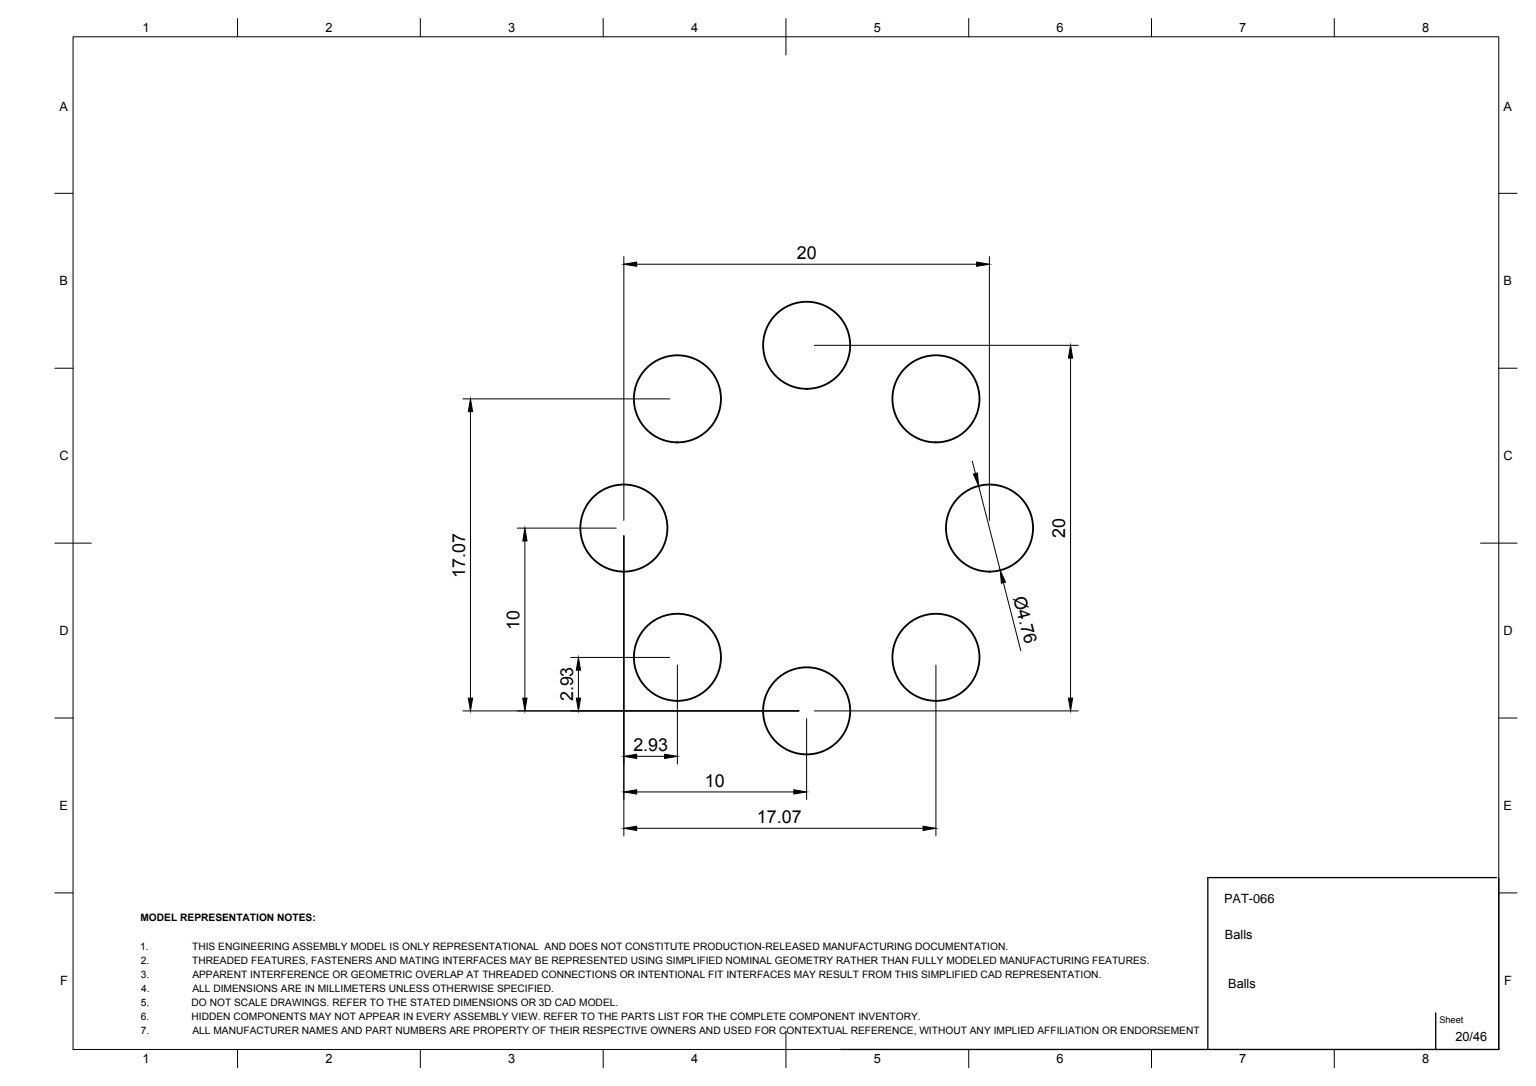
ISO-10303-21;
HEADER;
/* Generated by software containing ST-Developer
 * from STEP Tools, Inc. (www.steptools.com) 
 */

FILE_DESCRIPTION(
/* description */ ('Lever-operated bar clamp (toggle)'),
/* implementation_level */ '2;1');

FILE_NAME(
/* name */ 'Balls.step',
/* time_stamp */ '2026-10-28T03:25:02-07:00',
/* author */ (''),
/* organization */ (''),
/* preprocessor_version */ 'ST-DEVELOPER v20.2',
/* originating_system */ 'Autodesk Translation Framework v15.17.0.0',
/* authorisation */ '');

FILE_SCHEMA (('AUTOMOTIVE_DESIGN { 1 0 10303 214 3 1 1 }'));
ENDSEC;

DATA;
#10=MECHANICAL_DESIGN_GEOMETRIC_PRESENTATION_REPRESENTATION('',(#424,#425,#426,#427,#428,#429,#430,#431),#12413);
#287=SPHERICAL_SURFACE('',#7369,0.23815);
#288=SPHERICAL_SURFACE('',#7371,0.23815);
#289=SPHERICAL_SURFACE('',#7373,0.23815);
#290=SPHERICAL_SURFACE('',#7375,0.23815);
#291=SPHERICAL_SURFACE('',#7377,0.23815);
#292=SPHERICAL_SURFACE('',#7379,0.23815);
#293=SPHERICAL_SURFACE('',#7381,0.23815);
#294=SPHERICAL_SURFACE('',#7383,0.23815);
#348=SHAPE_REPRESENTATION_RELATIONSHIP('SRR','None',#12588,#386);
#386=ADVANCED_BREP_SHAPE_REPRESENTATION('',(#470,#471,#472,#473,#474,#475,
#476,#477),#12385);
#424=STYLED_ITEM('',(#12869),#470);
#425=STYLED_ITEM('',(#12869),#471);
#426=STYLED_ITEM('',(#12869),#472);
#427=STYLED_ITEM('',(#12869),#473);
#428=STYLED_ITEM('',(#12869),#474);
#429=STYLED_ITEM('',(#12869),#475);
#430=STYLED_ITEM('',(#12869),#476);
#431=STYLED_ITEM('',(#12869),#477);
#470=MANIFOLD_SOLID_BREP('Body1',#6584);
#471=MANIFOLD_SOLID_BREP('Body2',#6585);
#472=MANIFOLD_SOLID_BREP('Body3',#6586);
#473=MANIFOLD_SOLID_BREP('Body4',#6587);
#474=MANIFOLD_SOLID_BREP('Body5',#6588);
#475=MANIFOLD_SOLID_BREP('Body6',#6589);
#476=MANIFOLD_SOLID_BREP('Body7',#6590);
#477=MANIFOLD_SOLID_BREP('Body8',#6591);
#1055=FACE_OUTER_BOUND('',#1553,.T.);
#1056=FACE_OUTER_BOUND('',#1554,.T.);
#1057=FACE_OUTER_BOUND('',#1555,.T.);
#1058=FACE_OUTER_BOUND('',#1556,.T.);
#1059=FACE_OUTER_BOUND('',#1557,.T.);
#1060=FACE_OUTER_BOUND('',#1558,.T.);
#1061=FACE_OUTER_BOUND('',#1559,.T.);
#1062=FACE_OUTER_BOUND('',#1560,.T.);
#1553=EDGE_LOOP('',(#5109,#5110));
#1554=EDGE_LOOP('',(#5111,#5112));
#1555=EDGE_LOOP('',(#5113,#5114));
#1556=EDGE_LOOP('',(#5115,#5116));
#1557=EDGE_LOOP('',(#5117,#5118));
#1558=EDGE_LOOP('',(#5119,#5120));
#1559=EDGE_LOOP('',(#5121,#5122));
#1560=EDGE_LOOP('',(#5123,#5124));
#2878=CIRCLE('',#7370,0.23815);
#2879=CIRCLE('',#7372,0.23815);
#2880=CIRCLE('',#7374,0.23815);
#2881=CIRCLE('',#7376,0.23815);
#2882=CIRCLE('',#7378,0.23815);
#2883=CIRCLE('',#7380,0.23815);
#2884=CIRCLE('',#7382,0.23815);
#2885=CIRCLE('',#7384,0.23815);
#3301=VERTEX_POINT('',#10802);
#3302=VERTEX_POINT('',#10803);
#3303=VERTEX_POINT('',#10806);
#3304=VERTEX_POINT('',#10807);
#3305=VERTEX_POINT('',#10810);
#3306=VERTEX_POINT('',#10811);
#3307=VERTEX_POINT('',#10814);
#3308=VERTEX_POINT('',#10815);
#3309=VERTEX_POINT('',#10818);
#3310=VERTEX_POINT('',#10819);
#3311=VERTEX_POINT('',#10822);
#3312=VERTEX_POINT('',#10823);
#3313=VERTEX_POINT('',#10826);
#3314=VERTEX_POINT('',#10827);
#3315=VERTEX_POINT('',#10830);
#3316=VERTEX_POINT('',#10831);
#3959=EDGE_CURVE('',#3301,#3302,#2878,.T.);
#3960=EDGE_CURVE('',#3303,#3304,#2879,.T.);
#3961=EDGE_CURVE('',#3305,#3306,#2880,.T.);
#3962=EDGE_CURVE('',#3307,#3308,#2881,.T.);
#3963=EDGE_CURVE('',#3309,#3310,#2882,.T.);
#3964=EDGE_CURVE('',#3311,#3312,#2883,.T.);
#3965=EDGE_CURVE('',#3313,#3314,#2884,.T.);
#3966=EDGE_CURVE('',#3315,#3316,#2885,.T.);
#5109=ORIENTED_EDGE('',*,*,#3959,.T.);
#5110=ORIENTED_EDGE('',*,*,#3959,.F.);
#5111=ORIENTED_EDGE('',*,*,#3960,.T.);
#5112=ORIENTED_EDGE('',*,*,#3960,.F.);
#5113=ORIENTED_EDGE('',*,*,#3961,.T.);
#5114=ORIENTED_EDGE('',*,*,#3961,.F.);
#5115=ORIENTED_EDGE('',*,*,#3962,.T.);
#5116=ORIENTED_EDGE('',*,*,#3962,.F.);
#5117=ORIENTED_EDGE('',*,*,#3963,.T.);
#5118=ORIENTED_EDGE('',*,*,#3963,.F.);
#5119=ORIENTED_EDGE('',*,*,#3964,.T.);
#5120=ORIENTED_EDGE('',*,*,#3964,.F.);
#5121=ORIENTED_EDGE('',*,*,#3965,.T.);
#5122=ORIENTED_EDGE('',*,*,#3965,.F.);
#5123=ORIENTED_EDGE('',*,*,#3966,.T.);
#5124=ORIENTED_EDGE('',*,*,#3966,.F.);
#6330=ADVANCED_FACE('',(#1055),#287,.T.);
#6331=ADVANCED_FACE('',(#1056),#288,.T.);
#6332=ADVANCED_FACE('',(#1057),#289,.T.);
#6333=ADVANCED_FACE('',(#1058),#290,.T.);
#6334=ADVANCED_FACE('',(#1059),#291,.T.);
#6335=ADVANCED_FACE('',(#1060),#292,.T.);
#6336=ADVANCED_FACE('',(#1061),#293,.T.);
#6337=ADVANCED_FACE('',(#1062),#294,.T.);
#6584=CLOSED_SHELL('',(#6330));
#6585=CLOSED_SHELL('',(#6331));
#6586=CLOSED_SHELL('',(#6332));
#6587=CLOSED_SHELL('',(#6333));
#6588=CLOSED_SHELL('',(#6334));
#6589=CLOSED_SHELL('',(#6335));
#6590=CLOSED_SHELL('',(#6336));
#6591=CLOSED_SHELL('',(#6337));
#7368=AXIS2_PLACEMENT_3D('',#10800,#8751,#8752);
#7369=AXIS2_PLACEMENT_3D('',#10801,#8753,#8754);
#7370=AXIS2_PLACEMENT_3D('',#10804,#8755,#8756);
#7371=AXIS2_PLACEMENT_3D('',#10805,#8757,#8758);
#7372=AXIS2_PLACEMENT_3D('',#10808,#8759,#8760);
#7373=AXIS2_PLACEMENT_3D('',#10809,#8761,#8762);
#7374=AXIS2_PLACEMENT_3D('',#10812,#8763,#8764);
#7375=AXIS2_PLACEMENT_3D('',#10813,#8765,#8766);
#7376=AXIS2_PLACEMENT_3D('',#10816,#8767,#8768);
#7377=AXIS2_PLACEMENT_3D('',#10817,#8769,#8770);
#7378=AXIS2_PLACEMENT_3D('',#10820,#8771,#8772);
#7379=AXIS2_PLACEMENT_3D('',#10821,#8773,#8774);
#7380=AXIS2_PLACEMENT_3D('',#10824,#8775,#8776);
#7381=AXIS2_PLACEMENT_3D('',#10825,#8777,#8778);
#7382=AXIS2_PLACEMENT_3D('',#10828,#8779,#8780);
#7383=AXIS2_PLACEMENT_3D('',#10829,#8781,#8782);
#7384=AXIS2_PLACEMENT_3D('',#10832,#8783,#8784);
#8751=DIRECTION('axis',(0.,0.,1.));
#8752=DIRECTION('refdir',(1.,0.,0.));
#8753=DIRECTION('center_axis',(0.,0.,1.));
#8754=DIRECTION('ref_axis',(1.,0.,0.));
#8755=DIRECTION('center_axis',(1.22464679914735E-16,-1.,0.));
#8756=DIRECTION('ref_axis',(-1.,-1.22464679914735E-16,0.));
#8757=DIRECTION('center_axis',(0.707106781186548,0.,0.707106781186548));
#8758=DIRECTION('ref_axis',(0.707106781186548,0.,-0.707106781186548));
#8759=DIRECTION('center_axis',(8.65956056235494E-17,-1.,-8.65956056235493E-17));
#8760=DIRECTION('ref_axis',(-0.707106781186547,-1.22464679914735E-16,0.707106781186547));
#8761=DIRECTION('center_axis',(1.,0.,0.));
#8762=DIRECTION('ref_axis',(6.12323399573676E-17,0.,-1.));
#8763=DIRECTION('center_axis',(7.49879891330929E-33,-1.,-1.22464679914735E-16));
#8764=DIRECTION('ref_axis',(-6.12323399573676E-17,-1.22464679914735E-16,
1.));
#8765=DIRECTION('center_axis',(0.707106781186548,0.,-0.707106781186548));
#8766=DIRECTION('ref_axis',(-0.707106781186548,0.,-0.707106781186548));
#8767=DIRECTION('center_axis',(-8.65956056235493E-17,-1.,-8.65956056235494E-17));
#8768=DIRECTION('ref_axis',(0.707106781186547,-1.22464679914735E-16,0.707106781186547));
#8769=DIRECTION('center_axis',(0.,0.,-1.));
#8770=DIRECTION('ref_axis',(-1.,0.,-1.22464679914735E-16));
#8771=DIRECTION('center_axis',(-1.22464679914735E-16,-1.,-1.49975978266186E-32));
#8772=DIRECTION('ref_axis',(1.,-1.22464679914735E-16,1.22464679914735E-16));
#8773=DIRECTION('center_axis',(-0.707106781186547,0.,-0.707106781186548));
#8774=DIRECTION('ref_axis',(-0.707106781186548,0.,0.707106781186547));
#8775=DIRECTION('center_axis',(-8.65956056235493E-17,-1.,8.65956056235493E-17));
#8776=DIRECTION('ref_axis',(0.707106781186548,-1.22464679914735E-16,-0.707106781186547));
#8777=DIRECTION('center_axis',(-1.,0.,0.));
#8778=DIRECTION('ref_axis',(-1.83697019872103E-16,0.,1.));
#8779=DIRECTION('center_axis',(-2.24963967399279E-32,-1.,1.22464679914735E-16));
#8780=DIRECTION('ref_axis',(1.83697019872103E-16,-1.22464679914735E-16,
-1.));
#8781=DIRECTION('center_axis',(-0.707106781186548,0.,0.707106781186548));
#8782=DIRECTION('ref_axis',(0.707106781186547,0.,0.707106781186548));
#8783=DIRECTION('center_axis',(8.65956056235493E-17,-1.,8.65956056235493E-17));
#8784=DIRECTION('ref_axis',(-0.707106781186547,-1.22464679914735E-16,-0.707106781186548));
#10800=CARTESIAN_POINT('',(0.,0.,0.));
#10801=CARTESIAN_POINT('Origin',(1.,0.,0.));
#10802=CARTESIAN_POINT('',(1.,-1.78583896120461E-33,0.23815));
#10803=CARTESIAN_POINT('',(1.,-1.78583896120461E-33,-0.23815));
#10804=CARTESIAN_POINT('Origin',(1.,0.,0.));
#10805=CARTESIAN_POINT('Origin',(0.707106781186548,0.,-0.707106781186547));
#10806=CARTESIAN_POINT('',(0.875504261126124,-1.78583896120461E-33,-0.538709301246971));
#10807=CARTESIAN_POINT('',(0.538709301246971,-1.78583896120461E-33,-0.875504261126124));
#10808=CARTESIAN_POINT('Origin',(0.707106781186548,0.,-0.707106781186547));
#10809=CARTESIAN_POINT('Origin',(6.12323399573677E-17,0.,-1.));
#10810=CARTESIAN_POINT('',(0.23815,-1.78583896120461E-33,-1.));
#10811=CARTESIAN_POINT('',(-0.23815,-1.78583896120461E-33,-1.));
#10812=CARTESIAN_POINT('Origin',(6.12323399573677E-17,0.,-1.));
#10813=CARTESIAN_POINT('Origin',(-0.707106781186547,0.,-0.707106781186548));
#10814=CARTESIAN_POINT('',(-0.538709301246971,-1.78583896120461E-33,-0.875504261126124));
#10815=CARTESIAN_POINT('',(-0.875504261126124,-1.78583896120461E-33,-0.538709301246971));
#10816=CARTESIAN_POINT('Origin',(-0.707106781186547,0.,-0.707106781186548));
#10817=CARTESIAN_POINT('Origin',(-1.,0.,-1.22464679914735E-16));
#10818=CARTESIAN_POINT('',(-1.,-1.78583896120461E-33,-0.23815));
#10819=CARTESIAN_POINT('',(-1.,-1.78583896120461E-33,0.23815));
#10820=CARTESIAN_POINT('Origin',(-1.,0.,-1.22464679914735E-16));
#10821=CARTESIAN_POINT('Origin',(-0.707106781186548,0.,0.707106781186547));
#10822=CARTESIAN_POINT('',(-0.875504261126124,-7.94881478324376E-33,0.538709301246971));
#10823=CARTESIAN_POINT('',(-0.538709301246971,4.37713686083455E-33,0.875504261126124));
#10824=CARTESIAN_POINT('Origin',(-0.707106781186548,0.,0.707106781186547));
#10825=CARTESIAN_POINT('Origin',(-1.83697019872103E-16,0.,1.));
#10826=CARTESIAN_POINT('',(-0.23815,-1.78583896120461E-33,1.));
#10827=CARTESIAN_POINT('',(0.23815,-1.78583896120461E-33,1.));
#10828=CARTESIAN_POINT('Origin',(-1.83697019872103E-16,0.,1.));
#10829=CARTESIAN_POINT('Origin',(0.707106781186547,0.,0.707106781186548));
#10830=CARTESIAN_POINT('',(0.538709301246971,-4.86732687222419E-33,0.875504261126124));
#10831=CARTESIAN_POINT('',(0.875504261126124,1.29564894981497E-33,0.538709301246971));
#10832=CARTESIAN_POINT('Origin',(0.707106781186547,0.,0.707106781186548));
#12339=UNCERTAINTY_MEASURE_WITH_UNIT(LENGTH_MEASURE(0.001),#12414,
'DISTANCE_ACCURACY_VALUE',
'Maximum model space distance between geometric entities at asserted c
onnectivities');
#12367=UNCERTAINTY_MEASURE_WITH_UNIT(LENGTH_MEASURE(0.001),#12414,
'DISTANCE_ACCURACY_VALUE',
'Maximum model space distance between geometric entities at asserted c
onnectivities');
#12385=(
GEOMETRIC_REPRESENTATION_CONTEXT(3)
GLOBAL_UNCERTAINTY_ASSIGNED_CONTEXT((#12339))
GLOBAL_UNIT_ASSIGNED_CONTEXT((#12414,#12416,#12417))
REPRESENTATION_CONTEXT('','3D')
);
#12413=(
GEOMETRIC_REPRESENTATION_CONTEXT(3)
GLOBAL_UNCERTAINTY_ASSIGNED_CONTEXT((#12367))
GLOBAL_UNIT_ASSIGNED_CONTEXT((#12414,#12416,#12417))
REPRESENTATION_CONTEXT('','3D')
);
#12414=(
LENGTH_UNIT()
NAMED_UNIT(*)
SI_UNIT(.CENTI.,.METRE.)
);
#12416=(
NAMED_UNIT(*)
PLANE_ANGLE_UNIT()
SI_UNIT($,.RADIAN.)
);
#12417=(
NAMED_UNIT(*)
SI_UNIT($,.STERADIAN.)
SOLID_ANGLE_UNIT()
);
#12435=SHAPE_DEFINITION_REPRESENTATION(#12480,#12588);
#12480=PRODUCT_DEFINITION_SHAPE('',$,#12634);
#12588=SHAPE_REPRESENTATION('',(#7368),#12385);
#12616=PRODUCT_DEFINITION_CONTEXT('part definition',#12753,'design');
#12634=PRODUCT_DEFINITION('Balls','Balls',#12679,#12616);
#12679=PRODUCT_DEFINITION_FORMATION('',$,#12772);
#12753=APPLICATION_CONTEXT(
'Core Data for Automotive Mechanical Design Process');
#12754=PRODUCT_CONTEXT('part definition',#12753,'mechanical');
#12772=PRODUCT('Balls','Balls','Balls',(#12754));
#12863=COLOUR_RGB('Grey',0.48,0.52,0.57);
#12864=FILL_AREA_STYLE_COLOUR('',#12863);
#12865=FILL_AREA_STYLE('',(#12864));
#12866=SURFACE_STYLE_FILL_AREA(#12865);
#12867=SURFACE_SIDE_STYLE('',(#12866));
#12868=SURFACE_STYLE_USAGE(.BOTH.,#12867);
#12869=PRESENTATION_STYLE_ASSIGNMENT((#12868));
ENDSEC;
END-ISO-10303-21;
